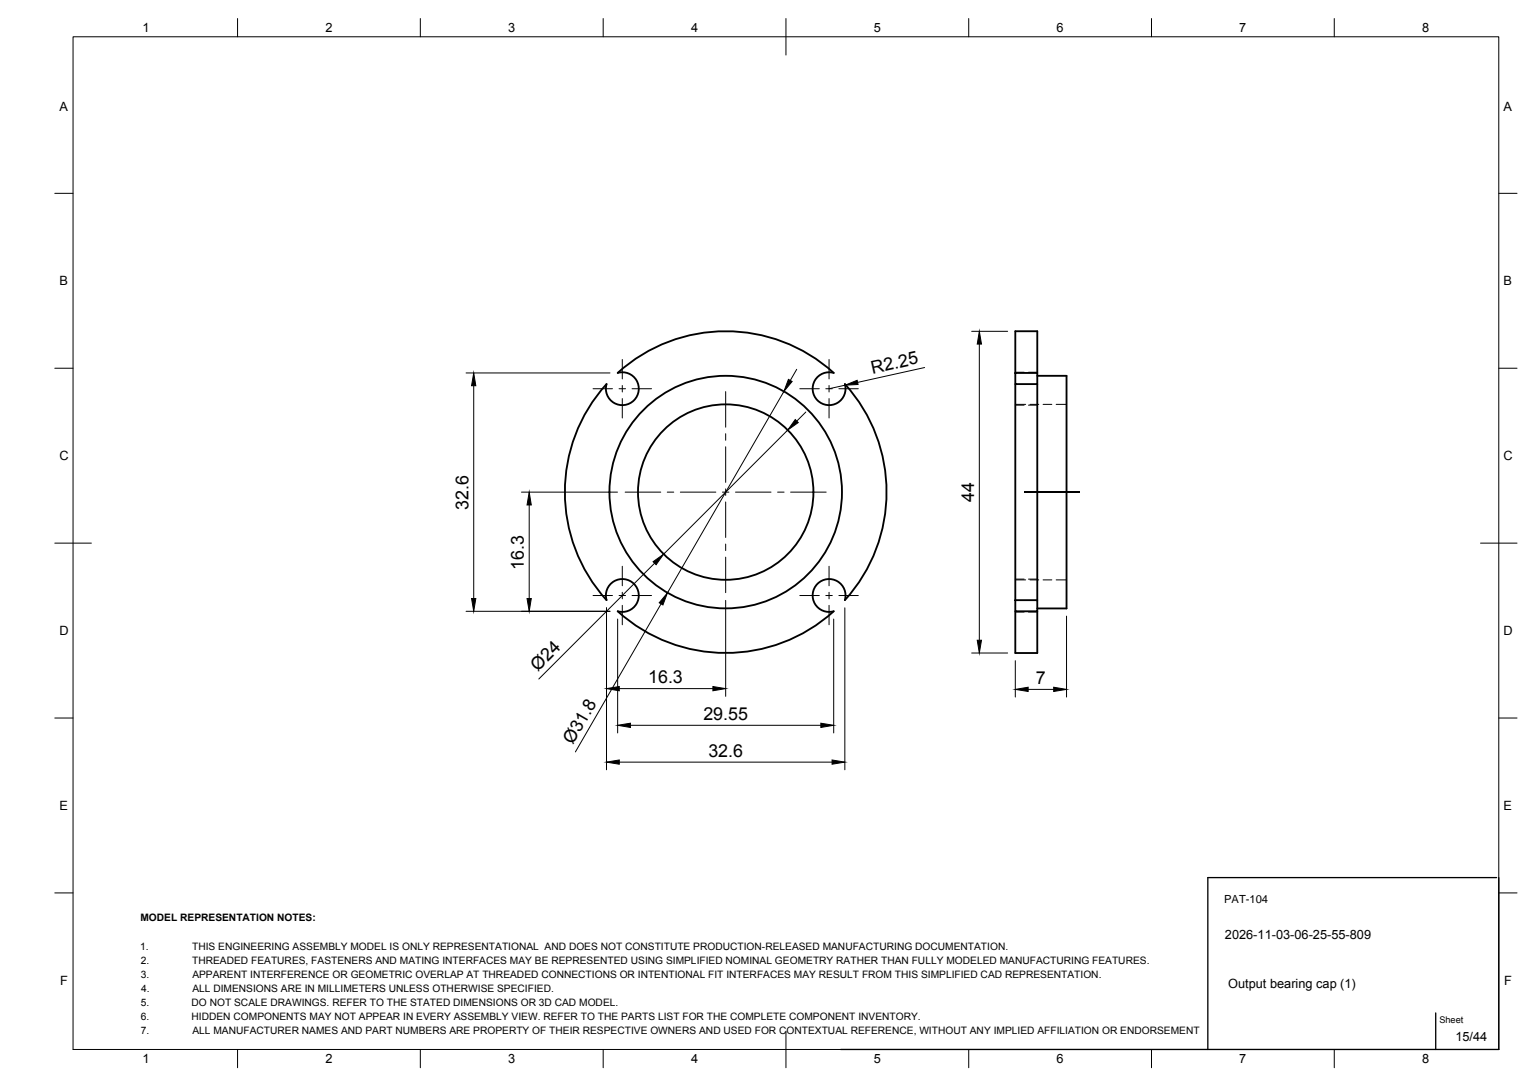
ISO-10303-21;
HEADER;
/* Generated by software containing ST-Developer
 * from STEP Tools, Inc. (www.steptools.com) 
 */

FILE_DESCRIPTION(
/* description */ ('Timing belt drive module 2 mm Pitch Timing 20T-40T'),

/* implementation_level */ '2;1');

FILE_NAME(
/* name */ 'Output bearing cap (1).step',
/* time_stamp */ '2026-10-28T03:25:12-07:00',
/* author */ (''),
/* organization */ (''),
/* preprocessor_version */ 'ST-DEVELOPER v20.2',
/* originating_system */ 'Autodesk Translation Framework v15.17.0.0',
/* authorisation */ '');

FILE_SCHEMA (('AUTOMOTIVE_DESIGN { 1 0 10303 214 3 1 1 }'));
ENDSEC;

DATA;
#10=MECHANICAL_DESIGN_GEOMETRIC_PRESENTATION_REPRESENTATION('',(#538),#17830);
#452=SHAPE_REPRESENTATION_RELATIONSHIP('SRR','None',#18022,#495);
#495=ADVANCED_BREP_SHAPE_REPRESENTATION('',(#596),#17797);
#538=STYLED_ITEM('',(#18317),#596);
#596=MANIFOLD_SOLID_BREP('Body1',#8995);
#704=FACE_BOUND('',#1698,.T.);
#705=FACE_BOUND('',#1705,.T.);
#706=FACE_BOUND('',#1708,.T.);
#844=PLANE('',#9836);
#845=PLANE('',#9852);
#846=PLANE('',#9856);
#1105=FACE_OUTER_BOUND('',#1693,.T.);
#1106=FACE_OUTER_BOUND('',#1694,.T.);
#1107=FACE_OUTER_BOUND('',#1695,.T.);
#1108=FACE_OUTER_BOUND('',#1696,.T.);
#1109=FACE_OUTER_BOUND('',#1697,.T.);
#1110=FACE_OUTER_BOUND('',#1699,.T.);
#1111=FACE_OUTER_BOUND('',#1700,.T.);
#1112=FACE_OUTER_BOUND('',#1701,.T.);
#1113=FACE_OUTER_BOUND('',#1702,.T.);
#1114=FACE_OUTER_BOUND('',#1703,.T.);
#1115=FACE_OUTER_BOUND('',#1704,.T.);
#1116=FACE_OUTER_BOUND('',#1706,.T.);
#1117=FACE_OUTER_BOUND('',#1707,.T.);
#1693=EDGE_LOOP('',(#6433,#6434,#6435,#6436));
#1694=EDGE_LOOP('',(#6437,#6438,#6439,#6440));
#1695=EDGE_LOOP('',(#6441,#6442,#6443,#6444));
#1696=EDGE_LOOP('',(#6445,#6446,#6447,#6448));
#1697=EDGE_LOOP('',(#6449,#6450,#6451,#6452,#6453,#6454,#6455,#6456));
#1698=EDGE_LOOP('',(#6457));
#1699=EDGE_LOOP('',(#6458,#6459,#6460,#6461));
#1700=EDGE_LOOP('',(#6462,#6463,#6464,#6465));
#1701=EDGE_LOOP('',(#6466,#6467,#6468,#6469));
#1702=EDGE_LOOP('',(#6470,#6471,#6472,#6473));
#1703=EDGE_LOOP('',(#6474,#6475,#6476,#6477));
#1704=EDGE_LOOP('',(#6478));
#1705=EDGE_LOOP('',(#6479));
#1706=EDGE_LOOP('',(#6480,#6481,#6482,#6483));
#1707=EDGE_LOOP('',(#6484,#6485,#6486,#6487,#6488,#6489,#6490,#6491));
#1708=EDGE_LOOP('',(#6492));
#2288=CIRCLE('',#9825,0.225);
#2289=CIRCLE('',#9826,0.225);
#2290=CIRCLE('',#9828,0.225);
#2291=CIRCLE('',#9829,0.225);
#2292=CIRCLE('',#9831,0.225);
#2293=CIRCLE('',#9832,0.225);
#2294=CIRCLE('',#9834,0.225);
#2295=CIRCLE('',#9835,0.225);
#2296=CIRCLE('',#9837,2.2);
#2297=CIRCLE('',#9838,2.2);
#2298=CIRCLE('',#9839,2.2);
#2299=CIRCLE('',#9840,2.2);
#2300=CIRCLE('',#9841,1.59);
#2301=CIRCLE('',#9843,2.2);
#2302=CIRCLE('',#9845,2.2);
#2303=CIRCLE('',#9847,2.2);
#2304=CIRCLE('',#9849,2.2);
#2305=CIRCLE('',#9851,1.59);
#2306=CIRCLE('',#9853,1.2);
#2307=CIRCLE('',#9855,1.2);
#2972=LINE('',#14586,#3450);
#2973=LINE('',#14590,#3451);
#2974=LINE('',#14595,#3452);
#2975=LINE('',#14599,#3453);
#2976=LINE('',#14604,#3454);
#2977=LINE('',#14608,#3455);
#2978=LINE('',#14613,#3456);
#2979=LINE('',#14617,#3457);
#2980=LINE('',#14636,#3458);
#2981=LINE('',#14644,#3459);
#3450=VECTOR('',#11609,1.);
#3451=VECTOR('',#11612,1.);
#3452=VECTOR('',#11617,1.);
#3453=VECTOR('',#11620,1.);
#3454=VECTOR('',#11625,1.);
#3455=VECTOR('',#11628,1.);
#3456=VECTOR('',#11633,1.);
#3457=VECTOR('',#11636,1.);
#3458=VECTOR('',#11669,1.59);
#3459=VECTOR('',#11680,1.2);
#3966=VERTEX_POINT('',#14584);
#3967=VERTEX_POINT('',#14585);
#3968=VERTEX_POINT('',#14587);
#3969=VERTEX_POINT('',#14589);
#3970=VERTEX_POINT('',#14593);
#3971=VERTEX_POINT('',#14594);
#3972=VERTEX_POINT('',#14596);
#3973=VERTEX_POINT('',#14598);
#3974=VERTEX_POINT('',#14602);
#3975=VERTEX_POINT('',#14603);
#3976=VERTEX_POINT('',#14605);
#3977=VERTEX_POINT('',#14607);
#3978=VERTEX_POINT('',#14611);
#3979=VERTEX_POINT('',#14612);
#3980=VERTEX_POINT('',#14614);
#3981=VERTEX_POINT('',#14616);
#3982=VERTEX_POINT('',#14624);
#3983=VERTEX_POINT('',#14635);
#3984=VERTEX_POINT('',#14639);
#3985=VERTEX_POINT('',#14642);
#4899=EDGE_CURVE('',#3966,#3967,#2972,.T.);
#4900=EDGE_CURVE('',#3968,#3966,#2288,.T.);
#4901=EDGE_CURVE('',#3969,#3968,#2973,.T.);
#4902=EDGE_CURVE('',#3967,#3969,#2289,.T.);
#4903=EDGE_CURVE('',#3970,#3971,#2974,.T.);
#4904=EDGE_CURVE('',#3972,#3970,#2290,.T.);
#4905=EDGE_CURVE('',#3973,#3972,#2975,.T.);
#4906=EDGE_CURVE('',#3971,#3973,#2291,.T.);
#4907=EDGE_CURVE('',#3974,#3975,#2976,.T.);
#4908=EDGE_CURVE('',#3976,#3974,#2292,.T.);
#4909=EDGE_CURVE('',#3977,#3976,#2977,.T.);
#4910=EDGE_CURVE('',#3975,#3977,#2293,.T.);
#4911=EDGE_CURVE('',#3978,#3979,#2978,.T.);
#4912=EDGE_CURVE('',#3980,#3978,#2294,.T.);
#4913=EDGE_CURVE('',#3981,#3980,#2979,.T.);
#4914=EDGE_CURVE('',#3979,#3981,#2295,.T.);
#4915=EDGE_CURVE('',#3980,#3966,#2296,.T.);
#4916=EDGE_CURVE('',#3976,#3978,#2297,.T.);
#4917=EDGE_CURVE('',#3972,#3974,#2298,.T.);
#4918=EDGE_CURVE('',#3968,#3970,#2299,.T.);
#4919=EDGE_CURVE('',#3982,#3982,#2300,.T.);
#4920=EDGE_CURVE('',#3977,#3979,#2301,.T.);
#4921=EDGE_CURVE('',#3973,#3975,#2302,.T.);
#4922=EDGE_CURVE('',#3981,#3967,#2303,.T.);
#4923=EDGE_CURVE('',#3969,#3971,#2304,.T.);
#4924=EDGE_CURVE('',#3982,#3983,#2980,.T.);
#4925=EDGE_CURVE('',#3983,#3983,#2305,.T.);
#4926=EDGE_CURVE('',#3984,#3984,#2306,.T.);
#4927=EDGE_CURVE('',#3985,#3985,#2307,.T.);
#4928=EDGE_CURVE('',#3985,#3984,#2981,.T.);
#6433=ORIENTED_EDGE('',*,*,#4899,.F.);
#6434=ORIENTED_EDGE('',*,*,#4900,.F.);
#6435=ORIENTED_EDGE('',*,*,#4901,.F.);
#6436=ORIENTED_EDGE('',*,*,#4902,.F.);
#6437=ORIENTED_EDGE('',*,*,#4903,.F.);
#6438=ORIENTED_EDGE('',*,*,#4904,.F.);
#6439=ORIENTED_EDGE('',*,*,#4905,.F.);
#6440=ORIENTED_EDGE('',*,*,#4906,.F.);
#6441=ORIENTED_EDGE('',*,*,#4907,.F.);
#6442=ORIENTED_EDGE('',*,*,#4908,.F.);
#6443=ORIENTED_EDGE('',*,*,#4909,.F.);
#6444=ORIENTED_EDGE('',*,*,#4910,.F.);
#6445=ORIENTED_EDGE('',*,*,#4911,.F.);
#6446=ORIENTED_EDGE('',*,*,#4912,.F.);
#6447=ORIENTED_EDGE('',*,*,#4913,.F.);
#6448=ORIENTED_EDGE('',*,*,#4914,.F.);
#6449=ORIENTED_EDGE('',*,*,#4900,.T.);
#6450=ORIENTED_EDGE('',*,*,#4915,.F.);
#6451=ORIENTED_EDGE('',*,*,#4912,.T.);
#6452=ORIENTED_EDGE('',*,*,#4916,.F.);
#6453=ORIENTED_EDGE('',*,*,#4908,.T.);
#6454=ORIENTED_EDGE('',*,*,#4917,.F.);
#6455=ORIENTED_EDGE('',*,*,#4904,.T.);
#6456=ORIENTED_EDGE('',*,*,#4918,.F.);
#6457=ORIENTED_EDGE('',*,*,#4919,.T.);
#6458=ORIENTED_EDGE('',*,*,#4909,.T.);
#6459=ORIENTED_EDGE('',*,*,#4916,.T.);
#6460=ORIENTED_EDGE('',*,*,#4911,.T.);
#6461=ORIENTED_EDGE('',*,*,#4920,.F.);
#6462=ORIENTED_EDGE('',*,*,#4905,.T.);
#6463=ORIENTED_EDGE('',*,*,#4917,.T.);
#6464=ORIENTED_EDGE('',*,*,#4907,.T.);
#6465=ORIENTED_EDGE('',*,*,#4921,.F.);
#6466=ORIENTED_EDGE('',*,*,#4899,.T.);
#6467=ORIENTED_EDGE('',*,*,#4922,.F.);
#6468=ORIENTED_EDGE('',*,*,#4913,.T.);
#6469=ORIENTED_EDGE('',*,*,#4915,.T.);
#6470=ORIENTED_EDGE('',*,*,#4901,.T.);
#6471=ORIENTED_EDGE('',*,*,#4918,.T.);
#6472=ORIENTED_EDGE('',*,*,#4903,.T.);
#6473=ORIENTED_EDGE('',*,*,#4923,.F.);
#6474=ORIENTED_EDGE('',*,*,#4919,.F.);
#6475=ORIENTED_EDGE('',*,*,#4924,.T.);
#6476=ORIENTED_EDGE('',*,*,#4925,.T.);
#6477=ORIENTED_EDGE('',*,*,#4924,.F.);
#6478=ORIENTED_EDGE('',*,*,#4925,.F.);
#6479=ORIENTED_EDGE('',*,*,#4926,.F.);
#6480=ORIENTED_EDGE('',*,*,#4927,.F.);
#6481=ORIENTED_EDGE('',*,*,#4928,.T.);
#6482=ORIENTED_EDGE('',*,*,#4926,.T.);
#6483=ORIENTED_EDGE('',*,*,#4928,.F.);
#6484=ORIENTED_EDGE('',*,*,#4902,.T.);
#6485=ORIENTED_EDGE('',*,*,#4923,.T.);
#6486=ORIENTED_EDGE('',*,*,#4906,.T.);
#6487=ORIENTED_EDGE('',*,*,#4921,.T.);
#6488=ORIENTED_EDGE('',*,*,#4910,.T.);
#6489=ORIENTED_EDGE('',*,*,#4920,.T.);
#6490=ORIENTED_EDGE('',*,*,#4914,.T.);
#6491=ORIENTED_EDGE('',*,*,#4922,.T.);
#6492=ORIENTED_EDGE('',*,*,#4927,.T.);
#8253=CYLINDRICAL_SURFACE('',#9824,0.225);
#8254=CYLINDRICAL_SURFACE('',#9827,0.225);
#8255=CYLINDRICAL_SURFACE('',#9830,0.225);
#8256=CYLINDRICAL_SURFACE('',#9833,0.225);
#8257=CYLINDRICAL_SURFACE('',#9842,2.2);
#8258=CYLINDRICAL_SURFACE('',#9844,2.2);
#8259=CYLINDRICAL_SURFACE('',#9846,2.2);
#8260=CYLINDRICAL_SURFACE('',#9848,2.2);
#8261=CYLINDRICAL_SURFACE('',#9850,1.59);
#8262=CYLINDRICAL_SURFACE('',#9854,1.2);
#8603=ADVANCED_FACE('',(#1105),#8253,.F.);
#8604=ADVANCED_FACE('',(#1106),#8254,.F.);
#8605=ADVANCED_FACE('',(#1107),#8255,.F.);
#8606=ADVANCED_FACE('',(#1108),#8256,.F.);
#8607=ADVANCED_FACE('',(#1109,#704),#844,.F.);
#8608=ADVANCED_FACE('',(#1110),#8257,.T.);
#8609=ADVANCED_FACE('',(#1111),#8258,.T.);
#8610=ADVANCED_FACE('',(#1112),#8259,.T.);
#8611=ADVANCED_FACE('',(#1113),#8260,.T.);
#8612=ADVANCED_FACE('',(#1114),#8261,.T.);
#8613=ADVANCED_FACE('',(#1115,#705),#845,.F.);
#8614=ADVANCED_FACE('',(#1116),#8262,.F.);
#8615=ADVANCED_FACE('',(#1117,#706),#846,.T.);
#8995=CLOSED_SHELL('',(#8603,#8604,#8605,#8606,#8607,#8608,#8609,#8610,
#8611,#8612,#8613,#8614,#8615));
#9823=AXIS2_PLACEMENT_3D('',#14582,#11605,#11606);
#9824=AXIS2_PLACEMENT_3D('',#14583,#11607,#11608);
#9825=AXIS2_PLACEMENT_3D('',#14588,#11610,#11611);
#9826=AXIS2_PLACEMENT_3D('',#14591,#11613,#11614);
#9827=AXIS2_PLACEMENT_3D('',#14592,#11615,#11616);
#9828=AXIS2_PLACEMENT_3D('',#14597,#11618,#11619);
#9829=AXIS2_PLACEMENT_3D('',#14600,#11621,#11622);
#9830=AXIS2_PLACEMENT_3D('',#14601,#11623,#11624);
#9831=AXIS2_PLACEMENT_3D('',#14606,#11626,#11627);
#9832=AXIS2_PLACEMENT_3D('',#14609,#11629,#11630);
#9833=AXIS2_PLACEMENT_3D('',#14610,#11631,#11632);
#9834=AXIS2_PLACEMENT_3D('',#14615,#11634,#11635);
#9835=AXIS2_PLACEMENT_3D('',#14618,#11637,#11638);
#9836=AXIS2_PLACEMENT_3D('',#14619,#11639,#11640);
#9837=AXIS2_PLACEMENT_3D('',#14620,#11641,#11642);
#9838=AXIS2_PLACEMENT_3D('',#14621,#11643,#11644);
#9839=AXIS2_PLACEMENT_3D('',#14622,#11645,#11646);
#9840=AXIS2_PLACEMENT_3D('',#14623,#11647,#11648);
#9841=AXIS2_PLACEMENT_3D('',#14625,#11649,#11650);
#9842=AXIS2_PLACEMENT_3D('',#14626,#11651,#11652);
#9843=AXIS2_PLACEMENT_3D('',#14627,#11653,#11654);
#9844=AXIS2_PLACEMENT_3D('',#14628,#11655,#11656);
#9845=AXIS2_PLACEMENT_3D('',#14629,#11657,#11658);
#9846=AXIS2_PLACEMENT_3D('',#14630,#11659,#11660);
#9847=AXIS2_PLACEMENT_3D('',#14631,#11661,#11662);
#9848=AXIS2_PLACEMENT_3D('',#14632,#11663,#11664);
#9849=AXIS2_PLACEMENT_3D('',#14633,#11665,#11666);
#9850=AXIS2_PLACEMENT_3D('',#14634,#11667,#11668);
#9851=AXIS2_PLACEMENT_3D('',#14637,#11670,#11671);
#9852=AXIS2_PLACEMENT_3D('',#14638,#11672,#11673);
#9853=AXIS2_PLACEMENT_3D('',#14640,#11674,#11675);
#9854=AXIS2_PLACEMENT_3D('',#14641,#11676,#11677);
#9855=AXIS2_PLACEMENT_3D('',#14643,#11678,#11679);
#9856=AXIS2_PLACEMENT_3D('',#14645,#11681,#11682);
#11605=DIRECTION('axis',(0.,0.,1.));
#11606=DIRECTION('refdir',(1.,0.,0.));
#11607=DIRECTION('center_axis',(0.,1.,0.));
#11608=DIRECTION('ref_axis',(0.707106781186546,0.,0.707106781186549));
#11609=DIRECTION('',(0.,1.,0.));
#11610=DIRECTION('center_axis',(0.,1.,0.));
#11611=DIRECTION('ref_axis',(1.,0.,0.));
#11612=DIRECTION('',(0.,-1.,0.));
#11613=DIRECTION('center_axis',(0.,-1.,0.));
#11614=DIRECTION('ref_axis',(1.,0.,0.));
#11615=DIRECTION('center_axis',(0.,1.,0.));
#11616=DIRECTION('ref_axis',(0.707106781186544,0.,-0.707106781186551));
#11617=DIRECTION('',(0.,1.,0.));
#11618=DIRECTION('center_axis',(0.,1.,0.));
#11619=DIRECTION('ref_axis',(1.,0.,0.));
#11620=DIRECTION('',(0.,-1.,0.));
#11621=DIRECTION('center_axis',(0.,-1.,0.));
#11622=DIRECTION('ref_axis',(1.,0.,0.));
#11623=DIRECTION('center_axis',(0.,1.,0.));
#11624=DIRECTION('ref_axis',(-0.707106781186548,0.,-0.707106781186547));
#11625=DIRECTION('',(0.,1.,0.));
#11626=DIRECTION('center_axis',(0.,1.,0.));
#11627=DIRECTION('ref_axis',(1.,0.,0.));
#11628=DIRECTION('',(0.,-1.,0.));
#11629=DIRECTION('center_axis',(0.,-1.,0.));
#11630=DIRECTION('ref_axis',(1.,0.,0.));
#11631=DIRECTION('center_axis',(0.,1.,0.));
#11632=DIRECTION('ref_axis',(-0.707106781186544,0.,0.707106781186551));
#11633=DIRECTION('',(0.,1.,0.));
#11634=DIRECTION('center_axis',(0.,1.,0.));
#11635=DIRECTION('ref_axis',(1.,0.,0.));
#11636=DIRECTION('',(0.,-1.,0.));
#11637=DIRECTION('center_axis',(0.,-1.,0.));
#11638=DIRECTION('ref_axis',(1.,0.,0.));
#11639=DIRECTION('center_axis',(0.,1.,0.));
#11640=DIRECTION('ref_axis',(1.,0.,0.));
#11641=DIRECTION('center_axis',(0.,1.,0.));
#11642=DIRECTION('ref_axis',(1.,0.,0.));
#11643=DIRECTION('center_axis',(0.,1.,0.));
#11644=DIRECTION('ref_axis',(1.,0.,0.));
#11645=DIRECTION('center_axis',(0.,1.,0.));
#11646=DIRECTION('ref_axis',(1.,0.,0.));
#11647=DIRECTION('center_axis',(0.,1.,0.));
#11648=DIRECTION('ref_axis',(1.,0.,0.));
#11649=DIRECTION('center_axis',(0.,1.,0.));
#11650=DIRECTION('ref_axis',(1.,0.,0.));
#11651=DIRECTION('center_axis',(0.,1.,0.));
#11652=DIRECTION('ref_axis',(1.,0.,0.));
#11653=DIRECTION('center_axis',(0.,1.,0.));
#11654=DIRECTION('ref_axis',(1.,0.,0.));
#11655=DIRECTION('center_axis',(0.,1.,0.));
#11656=DIRECTION('ref_axis',(1.,0.,0.));
#11657=DIRECTION('center_axis',(0.,1.,0.));
#11658=DIRECTION('ref_axis',(1.,0.,0.));
#11659=DIRECTION('center_axis',(0.,1.,0.));
#11660=DIRECTION('ref_axis',(1.,0.,0.));
#11661=DIRECTION('center_axis',(0.,1.,0.));
#11662=DIRECTION('ref_axis',(1.,0.,0.));
#11663=DIRECTION('center_axis',(0.,1.,0.));
#11664=DIRECTION('ref_axis',(-1.,0.,-1.01064309961486E-15));
#11665=DIRECTION('center_axis',(0.,1.,0.));
#11666=DIRECTION('ref_axis',(1.,0.,0.));
#11667=DIRECTION('center_axis',(0.,1.,0.));
#11668=DIRECTION('ref_axis',(1.,0.,0.));
#11669=DIRECTION('',(0.,-1.,0.));
#11670=DIRECTION('center_axis',(0.,1.,0.));
#11671=DIRECTION('ref_axis',(1.,0.,0.));
#11672=DIRECTION('center_axis',(0.,1.,0.));
#11673=DIRECTION('ref_axis',(1.,0.,0.));
#11674=DIRECTION('center_axis',(0.,-1.,0.));
#11675=DIRECTION('ref_axis',(1.,0.,0.));
#11676=DIRECTION('center_axis',(0.,1.,0.));
#11677=DIRECTION('ref_axis',(1.,0.,0.));
#11678=DIRECTION('center_axis',(0.,-1.,0.));
#11679=DIRECTION('ref_axis',(1.,0.,0.));
#11680=DIRECTION('',(0.,-1.,0.));
#11681=DIRECTION('center_axis',(0.,1.,0.));
#11682=DIRECTION('ref_axis',(1.,0.,0.));
#14582=CARTESIAN_POINT('',(0.,0.,0.));
#14583=CARTESIAN_POINT('Origin',(5.55669646780806,1.7,5.58578643762691));
#14584=CARTESIAN_POINT('',(5.49357471024299,1.8,5.36982198749241));
#14585=CARTESIAN_POINT('',(5.49357471024299,2.1,5.36982198749241));
#14586=CARTESIAN_POINT('',(5.49357471024299,1.7,5.36982198749241));
#14587=CARTESIAN_POINT('',(5.34073201767356,1.8,5.52266468006184));
#14588=CARTESIAN_POINT('Origin',(5.55669646780806,1.8,5.58578643762691));
#14589=CARTESIAN_POINT('',(5.34073201767356,2.1,5.52266468006184));
#14590=CARTESIAN_POINT('',(5.34073201767356,1.7,5.52266468006184));
#14591=CARTESIAN_POINT('Origin',(5.55669646780806,2.1,5.58578643762691));
#14592=CARTESIAN_POINT('Origin',(5.55669646780806,1.7,8.4142135623731));
#14593=CARTESIAN_POINT('',(5.34073201767356,1.8,8.47733531993816));
#14594=CARTESIAN_POINT('',(5.34073201767356,2.1,8.47733531993816));
#14595=CARTESIAN_POINT('',(5.34073201767356,1.7,8.47733531993816));
#14596=CARTESIAN_POINT('',(5.493574710243,1.8,8.6301780125076));
#14597=CARTESIAN_POINT('Origin',(5.55669646780806,1.8,8.4142135623731));
#14598=CARTESIAN_POINT('',(5.493574710243,2.1,8.6301780125076));
#14599=CARTESIAN_POINT('',(5.493574710243,1.7,8.6301780125076));
#14600=CARTESIAN_POINT('Origin',(5.55669646780806,2.1,8.4142135623731));
#14601=CARTESIAN_POINT('Origin',(8.38512359255425,1.7,8.4142135623731));
#14602=CARTESIAN_POINT('',(8.44824535011931,1.8,8.6301780125076));
#14603=CARTESIAN_POINT('',(8.44824535011931,2.1,8.6301780125076));
#14604=CARTESIAN_POINT('',(8.44824535011932,1.7,8.6301780125076));
#14605=CARTESIAN_POINT('',(8.60108804268875,1.8,8.47733531993816));
#14606=CARTESIAN_POINT('Origin',(8.38512359255425,1.8,8.4142135623731));
#14607=CARTESIAN_POINT('',(8.60108804268875,2.1,8.47733531993816));
#14608=CARTESIAN_POINT('',(8.60108804268875,1.7,8.47733531993816));
#14609=CARTESIAN_POINT('Origin',(8.38512359255425,2.1,8.4142135623731));
#14610=CARTESIAN_POINT('Origin',(8.38512359255425,1.7,5.58578643762691));
#14611=CARTESIAN_POINT('',(8.60108804268875,1.8,5.52266468006184));
#14612=CARTESIAN_POINT('',(8.60108804268875,2.1,5.52266468006184));
#14613=CARTESIAN_POINT('',(8.60108804268875,1.7,5.52266468006184));
#14614=CARTESIAN_POINT('',(8.44824535011932,1.8,5.36982198749241));
#14615=CARTESIAN_POINT('Origin',(8.38512359255425,1.8,5.58578643762691));
#14616=CARTESIAN_POINT('',(8.44824535011932,2.1,5.36982198749241));
#14617=CARTESIAN_POINT('',(8.44824535011932,1.7,5.36982198749241));
#14618=CARTESIAN_POINT('Origin',(8.38512359255425,2.1,5.58578643762691));
#14619=CARTESIAN_POINT('Origin',(6.97091003018116,1.8,7.));
#14620=CARTESIAN_POINT('Origin',(6.97091003018116,1.8,7.));
#14621=CARTESIAN_POINT('Origin',(6.97091003018116,1.8,7.));
#14622=CARTESIAN_POINT('Origin',(6.97091003018116,1.8,7.));
#14623=CARTESIAN_POINT('Origin',(6.97091003018116,1.8,7.));
#14624=CARTESIAN_POINT('',(5.38091003018116,1.8,7.));
#14625=CARTESIAN_POINT('Origin',(6.97091003018116,1.8,7.));
#14626=CARTESIAN_POINT('Origin',(6.97091003018116,1.8,7.));
#14627=CARTESIAN_POINT('Origin',(6.97091003018116,2.1,7.));
#14628=CARTESIAN_POINT('Origin',(6.97091003018116,1.8,7.));
#14629=CARTESIAN_POINT('Origin',(6.97091003018116,2.1,7.));
#14630=CARTESIAN_POINT('Origin',(6.97091003018116,1.8,7.));
#14631=CARTESIAN_POINT('Origin',(6.97091003018116,2.1,7.));
#14632=CARTESIAN_POINT('Origin',(6.97091003018116,1.8,7.));
#14633=CARTESIAN_POINT('Origin',(6.97091003018116,2.1,7.));
#14634=CARTESIAN_POINT('Origin',(6.97091003018116,1.4,7.));
#14635=CARTESIAN_POINT('',(5.38091003018116,1.4,7.));
#14636=CARTESIAN_POINT('',(5.38091003018116,1.4,7.));
#14637=CARTESIAN_POINT('Origin',(6.97091003018116,1.4,7.));
#14638=CARTESIAN_POINT('Origin',(6.97091003018116,1.4,7.));
#14639=CARTESIAN_POINT('',(5.77091003018116,1.4,7.));
#14640=CARTESIAN_POINT('Origin',(6.97091003018116,1.4,7.));
#14641=CARTESIAN_POINT('Origin',(6.97091003018116,1.8,7.));
#14642=CARTESIAN_POINT('',(5.77091003018116,2.1,7.));
#14643=CARTESIAN_POINT('Origin',(6.97091003018116,2.1,7.));
#14644=CARTESIAN_POINT('',(5.77091003018116,1.8,7.));
#14645=CARTESIAN_POINT('Origin',(6.97091003018116,2.1,7.));
#17747=UNCERTAINTY_MEASURE_WITH_UNIT(LENGTH_MEASURE(0.001),#17831,
'DISTANCE_ACCURACY_VALUE',
'Maximum model space distance between geometric entities at asserted c
onnectivities');
#17780=UNCERTAINTY_MEASURE_WITH_UNIT(LENGTH_MEASURE(0.001),#17831,
'DISTANCE_ACCURACY_VALUE',
'Maximum model space distance between geometric entities at asserted c
onnectivities');
#17797=(
GEOMETRIC_REPRESENTATION_CONTEXT(3)
GLOBAL_UNCERTAINTY_ASSIGNED_CONTEXT((#17747))
GLOBAL_UNIT_ASSIGNED_CONTEXT((#17831,#17833,#17834))
REPRESENTATION_CONTEXT('','3D')
);
#17830=(
GEOMETRIC_REPRESENTATION_CONTEXT(3)
GLOBAL_UNCERTAINTY_ASSIGNED_CONTEXT((#17780))
GLOBAL_UNIT_ASSIGNED_CONTEXT((#17831,#17833,#17834))
REPRESENTATION_CONTEXT('','3D')
);
#17831=(
LENGTH_UNIT()
NAMED_UNIT(*)
SI_UNIT(.CENTI.,.METRE.)
);
#17833=(
NAMED_UNIT(*)
PLANE_ANGLE_UNIT()
SI_UNIT($,.RADIAN.)
);
#17834=(
NAMED_UNIT(*)
SI_UNIT($,.STERADIAN.)
SOLID_ANGLE_UNIT()
);
#17851=SHAPE_DEFINITION_REPRESENTATION(#17900,#18022);
#17900=PRODUCT_DEFINITION_SHAPE('',$,#18072);
#18022=SHAPE_REPRESENTATION('',(#9823),#17797);
#18055=PRODUCT_DEFINITION_CONTEXT('part definition',#18204,'design');
#18072=PRODUCT_DEFINITION('Output bearing cap (1)',
'Output bearing cap (1)',#18121,#18055);
#18121=PRODUCT_DEFINITION_FORMATION('',$,#18222);
#18204=APPLICATION_CONTEXT(
'Core Data for Automotive Mechanical Design Process');
#18205=PRODUCT_CONTEXT('part definition',#18204,'mechanical');
#18222=PRODUCT('Output bearing cap (1)','Output bearing cap (1)',
'Output bearing cap (1)',(#18205));
#18311=COLOUR_RGB('Grey',0.48,0.52,0.57);
#18312=FILL_AREA_STYLE_COLOUR('',#18311);
#18313=FILL_AREA_STYLE('',(#18312));
#18314=SURFACE_STYLE_FILL_AREA(#18313);
#18315=SURFACE_SIDE_STYLE('',(#18314));
#18316=SURFACE_STYLE_USAGE(.BOTH.,#18315);
#18317=PRESENTATION_STYLE_ASSIGNMENT((#18316));
ENDSEC;
END-ISO-10303-21;
